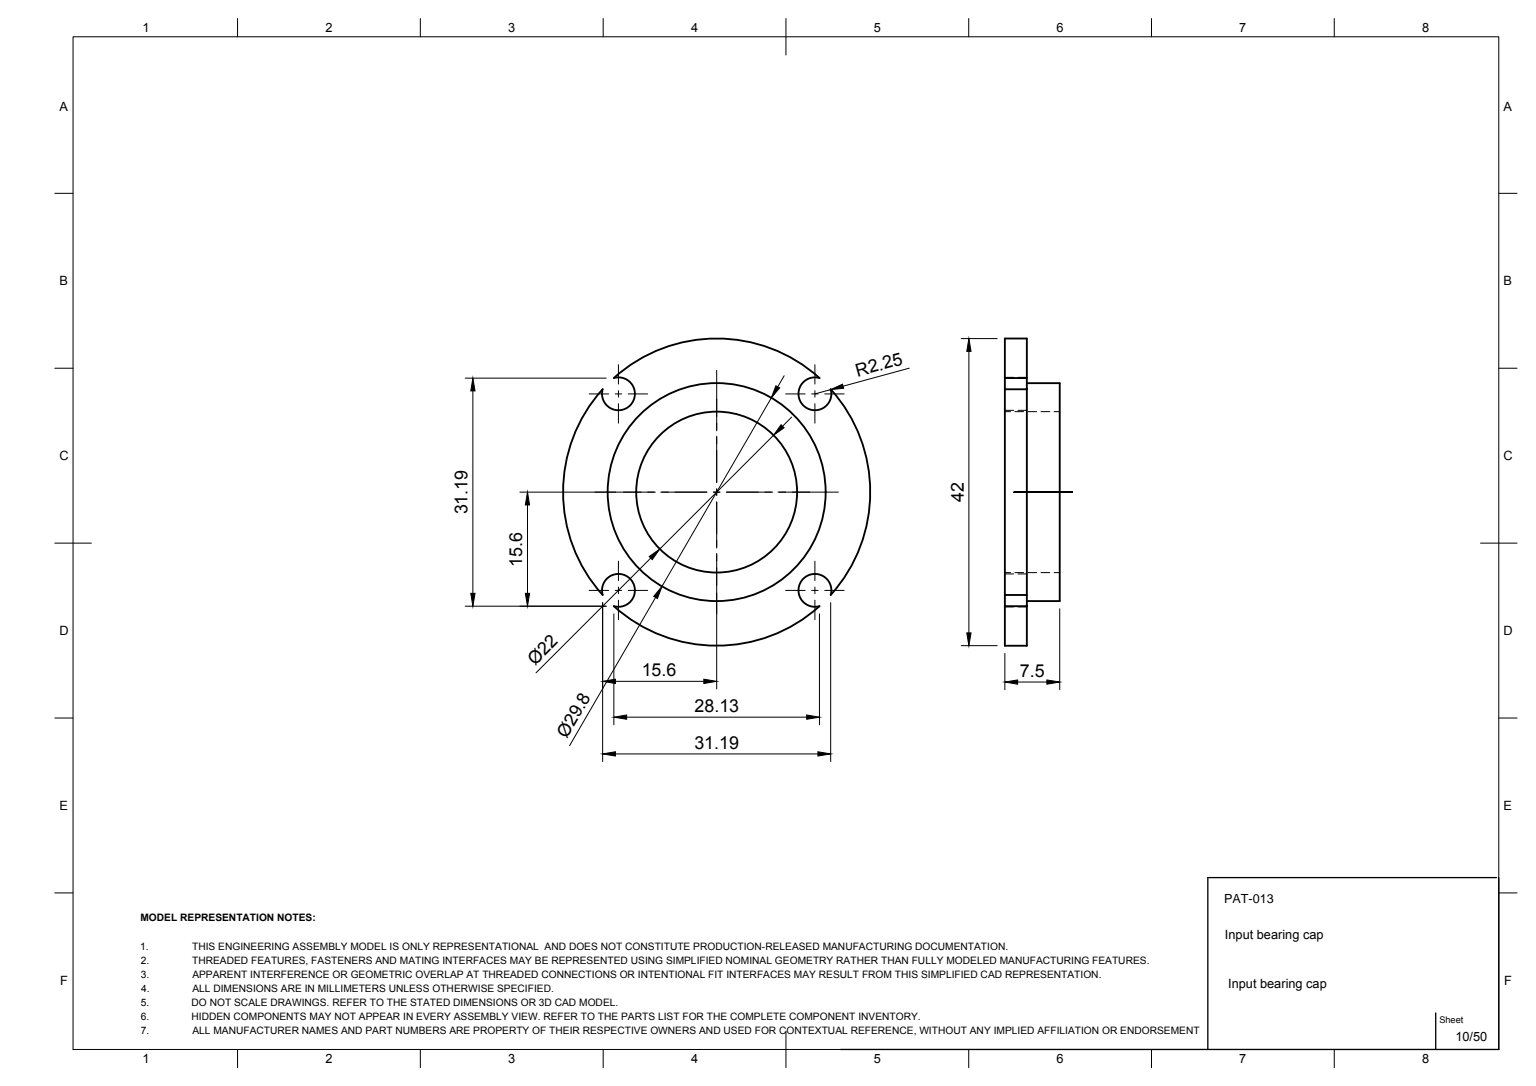
ISO-10303-21;
HEADER;
/* Generated by software containing ST-Developer
 * from STEP Tools, Inc. (www.steptools.com) 
 */

FILE_DESCRIPTION(
/* description */ ('Belt-driven linear axis on 2020 extrusion'),
/* implementation_level */ '2;1');

FILE_NAME(
/* name */ 'Input bearing cap.step',
/* time_stamp */ '2026-10-28T03:26:09-07:00',
/* author */ (''),
/* organization */ (''),
/* preprocessor_version */ 'ST-DEVELOPER v20.2',
/* originating_system */ 'Autodesk Translation Framework v15.17.0.0',
/* authorisation */ '');

FILE_SCHEMA (('AUTOMOTIVE_DESIGN { 1 0 10303 214 3 1 1 }'));
ENDSEC;

DATA;
#10=MECHANICAL_DESIGN_GEOMETRIC_PRESENTATION_REPRESENTATION('',(#617),#20096);
#523=SHAPE_REPRESENTATION_RELATIONSHIP('SRR','None',#20319,#569);
#569=ADVANCED_BREP_SHAPE_REPRESENTATION('',(#673),#20050);
#617=STYLED_ITEM('',(#20650),#673);
#673=MANIFOLD_SOLID_BREP('Body1',#10930);
#762=FACE_BOUND('',#2010,.T.);
#763=FACE_BOUND('',#2017,.T.);
#764=FACE_BOUND('',#2020,.T.);
#947=PLANE('',#11661);
#948=PLANE('',#11678);
#949=PLANE('',#11681);
#1339=FACE_OUTER_BOUND('',#2005,.T.);
#1340=FACE_OUTER_BOUND('',#2006,.T.);
#1341=FACE_OUTER_BOUND('',#2007,.T.);
#1342=FACE_OUTER_BOUND('',#2008,.T.);
#1343=FACE_OUTER_BOUND('',#2009,.T.);
#1344=FACE_OUTER_BOUND('',#2011,.T.);
#1345=FACE_OUTER_BOUND('',#2012,.T.);
#1346=FACE_OUTER_BOUND('',#2013,.T.);
#1347=FACE_OUTER_BOUND('',#2014,.T.);
#1348=FACE_OUTER_BOUND('',#2015,.T.);
#1349=FACE_OUTER_BOUND('',#2016,.T.);
#1350=FACE_OUTER_BOUND('',#2018,.T.);
#1351=FACE_OUTER_BOUND('',#2019,.T.);
#2005=EDGE_LOOP('',(#7607,#7608,#7609,#7610));
#2006=EDGE_LOOP('',(#7611,#7612,#7613,#7614));
#2007=EDGE_LOOP('',(#7615,#7616,#7617,#7618));
#2008=EDGE_LOOP('',(#7619,#7620,#7621,#7622));
#2009=EDGE_LOOP('',(#7623,#7624,#7625,#7626,#7627,#7628,#7629,#7630));
#2010=EDGE_LOOP('',(#7631));
#2011=EDGE_LOOP('',(#7632,#7633,#7634,#7635));
#2012=EDGE_LOOP('',(#7636,#7637,#7638,#7639));
#2013=EDGE_LOOP('',(#7640,#7641,#7642,#7643));
#2014=EDGE_LOOP('',(#7644,#7645,#7646,#7647));
#2015=EDGE_LOOP('',(#7648,#7649,#7650,#7651));
#2016=EDGE_LOOP('',(#7652));
#2017=EDGE_LOOP('',(#7653));
#2018=EDGE_LOOP('',(#7654,#7655,#7656,#7657));
#2019=EDGE_LOOP('',(#7658,#7659,#7660,#7661,#7662,#7663,#7664,#7665));
#2020=EDGE_LOOP('',(#7666));
#2780=LINE('',#16627,#3637);
#2781=LINE('',#16631,#3638);
#2782=LINE('',#16636,#3639);
#2783=LINE('',#16640,#3640);
#2784=LINE('',#16645,#3641);
#2785=LINE('',#16649,#3642);
#2786=LINE('',#16654,#3643);
#2787=LINE('',#16658,#3644);
#2788=LINE('',#16679,#3645);
#2789=LINE('',#16685,#3646);
#3637=VECTOR('',#13220,1.);
#3638=VECTOR('',#13223,1.);
#3639=VECTOR('',#13228,1.);
#3640=VECTOR('',#13231,1.);
#3641=VECTOR('',#13236,1.);
#3642=VECTOR('',#13239,1.);
#3643=VECTOR('',#13244,1.);
#3644=VECTOR('',#13247,1.);
#3645=VECTOR('',#13282,1.49);
#3646=VECTOR('',#13291,1.1);
#4441=CIRCLE('',#11650,0.225);
#4442=CIRCLE('',#11651,0.225);
#4443=CIRCLE('',#11653,0.225);
#4444=CIRCLE('',#11654,0.225);
#4445=CIRCLE('',#11656,0.225);
#4446=CIRCLE('',#11657,0.225);
#4447=CIRCLE('',#11659,0.225);
#4448=CIRCLE('',#11660,0.225);
#4449=CIRCLE('',#11662,2.1);
#4450=CIRCLE('',#11663,2.1);
#4451=CIRCLE('',#11664,2.1);
#4452=CIRCLE('',#11665,2.1);
#4453=CIRCLE('',#11666,1.1);
#4454=CIRCLE('',#11668,2.1);
#4455=CIRCLE('',#11670,2.1);
#4456=CIRCLE('',#11672,2.1);
#4457=CIRCLE('',#11674,2.1);
#4458=CIRCLE('',#11676,1.49);
#4459=CIRCLE('',#11677,1.49);
#4460=CIRCLE('',#11679,1.1);
#5010=VERTEX_POINT('',#16625);
#5011=VERTEX_POINT('',#16626);
#5012=VERTEX_POINT('',#16628);
#5013=VERTEX_POINT('',#16630);
#5014=VERTEX_POINT('',#16634);
#5015=VERTEX_POINT('',#16635);
#5016=VERTEX_POINT('',#16637);
#5017=VERTEX_POINT('',#16639);
#5018=VERTEX_POINT('',#16643);
#5019=VERTEX_POINT('',#16644);
#5020=VERTEX_POINT('',#16646);
#5021=VERTEX_POINT('',#16648);
#5022=VERTEX_POINT('',#16652);
#5023=VERTEX_POINT('',#16653);
#5024=VERTEX_POINT('',#16655);
#5025=VERTEX_POINT('',#16657);
#5026=VERTEX_POINT('',#16665);
#5027=VERTEX_POINT('',#16676);
#5028=VERTEX_POINT('',#16678);
#5029=VERTEX_POINT('',#16682);
#6018=EDGE_CURVE('',#5010,#5011,#2780,.T.);
#6019=EDGE_CURVE('',#5012,#5010,#4441,.T.);
#6020=EDGE_CURVE('',#5013,#5012,#2781,.T.);
#6021=EDGE_CURVE('',#5011,#5013,#4442,.T.);
#6022=EDGE_CURVE('',#5014,#5015,#2782,.T.);
#6023=EDGE_CURVE('',#5016,#5014,#4443,.T.);
#6024=EDGE_CURVE('',#5017,#5016,#2783,.T.);
#6025=EDGE_CURVE('',#5015,#5017,#4444,.T.);
#6026=EDGE_CURVE('',#5018,#5019,#2784,.T.);
#6027=EDGE_CURVE('',#5020,#5018,#4445,.T.);
#6028=EDGE_CURVE('',#5021,#5020,#2785,.T.);
#6029=EDGE_CURVE('',#5019,#5021,#4446,.T.);
#6030=EDGE_CURVE('',#5022,#5023,#2786,.T.);
#6031=EDGE_CURVE('',#5024,#5022,#4447,.T.);
#6032=EDGE_CURVE('',#5025,#5024,#2787,.T.);
#6033=EDGE_CURVE('',#5023,#5025,#4448,.T.);
#6034=EDGE_CURVE('',#5024,#5010,#4449,.T.);
#6035=EDGE_CURVE('',#5020,#5022,#4450,.T.);
#6036=EDGE_CURVE('',#5016,#5018,#4451,.T.);
#6037=EDGE_CURVE('',#5012,#5014,#4452,.T.);
#6038=EDGE_CURVE('',#5026,#5026,#4453,.T.);
#6039=EDGE_CURVE('',#5021,#5023,#4454,.T.);
#6040=EDGE_CURVE('',#5017,#5019,#4455,.T.);
#6041=EDGE_CURVE('',#5025,#5011,#4456,.T.);
#6042=EDGE_CURVE('',#5013,#5015,#4457,.T.);
#6043=EDGE_CURVE('',#5027,#5027,#4458,.T.);
#6044=EDGE_CURVE('',#5027,#5028,#2788,.T.);
#6045=EDGE_CURVE('',#5028,#5028,#4459,.T.);
#6046=EDGE_CURVE('',#5029,#5029,#4460,.T.);
#6047=EDGE_CURVE('',#5029,#5026,#2789,.T.);
#7607=ORIENTED_EDGE('',*,*,#6018,.F.);
#7608=ORIENTED_EDGE('',*,*,#6019,.F.);
#7609=ORIENTED_EDGE('',*,*,#6020,.F.);
#7610=ORIENTED_EDGE('',*,*,#6021,.F.);
#7611=ORIENTED_EDGE('',*,*,#6022,.F.);
#7612=ORIENTED_EDGE('',*,*,#6023,.F.);
#7613=ORIENTED_EDGE('',*,*,#6024,.F.);
#7614=ORIENTED_EDGE('',*,*,#6025,.F.);
#7615=ORIENTED_EDGE('',*,*,#6026,.F.);
#7616=ORIENTED_EDGE('',*,*,#6027,.F.);
#7617=ORIENTED_EDGE('',*,*,#6028,.F.);
#7618=ORIENTED_EDGE('',*,*,#6029,.F.);
#7619=ORIENTED_EDGE('',*,*,#6030,.F.);
#7620=ORIENTED_EDGE('',*,*,#6031,.F.);
#7621=ORIENTED_EDGE('',*,*,#6032,.F.);
#7622=ORIENTED_EDGE('',*,*,#6033,.F.);
#7623=ORIENTED_EDGE('',*,*,#6019,.T.);
#7624=ORIENTED_EDGE('',*,*,#6034,.F.);
#7625=ORIENTED_EDGE('',*,*,#6031,.T.);
#7626=ORIENTED_EDGE('',*,*,#6035,.F.);
#7627=ORIENTED_EDGE('',*,*,#6027,.T.);
#7628=ORIENTED_EDGE('',*,*,#6036,.F.);
#7629=ORIENTED_EDGE('',*,*,#6023,.T.);
#7630=ORIENTED_EDGE('',*,*,#6037,.F.);
#7631=ORIENTED_EDGE('',*,*,#6038,.F.);
#7632=ORIENTED_EDGE('',*,*,#6028,.T.);
#7633=ORIENTED_EDGE('',*,*,#6035,.T.);
#7634=ORIENTED_EDGE('',*,*,#6030,.T.);
#7635=ORIENTED_EDGE('',*,*,#6039,.F.);
#7636=ORIENTED_EDGE('',*,*,#6024,.T.);
#7637=ORIENTED_EDGE('',*,*,#6036,.T.);
#7638=ORIENTED_EDGE('',*,*,#6026,.T.);
#7639=ORIENTED_EDGE('',*,*,#6040,.F.);
#7640=ORIENTED_EDGE('',*,*,#6018,.T.);
#7641=ORIENTED_EDGE('',*,*,#6041,.F.);
#7642=ORIENTED_EDGE('',*,*,#6032,.T.);
#7643=ORIENTED_EDGE('',*,*,#6034,.T.);
#7644=ORIENTED_EDGE('',*,*,#6020,.T.);
#7645=ORIENTED_EDGE('',*,*,#6037,.T.);
#7646=ORIENTED_EDGE('',*,*,#6022,.T.);
#7647=ORIENTED_EDGE('',*,*,#6042,.F.);
#7648=ORIENTED_EDGE('',*,*,#6043,.F.);
#7649=ORIENTED_EDGE('',*,*,#6044,.T.);
#7650=ORIENTED_EDGE('',*,*,#6045,.F.);
#7651=ORIENTED_EDGE('',*,*,#6044,.F.);
#7652=ORIENTED_EDGE('',*,*,#6043,.T.);
#7653=ORIENTED_EDGE('',*,*,#6046,.T.);
#7654=ORIENTED_EDGE('',*,*,#6046,.F.);
#7655=ORIENTED_EDGE('',*,*,#6047,.T.);
#7656=ORIENTED_EDGE('',*,*,#6038,.T.);
#7657=ORIENTED_EDGE('',*,*,#6047,.F.);
#7658=ORIENTED_EDGE('',*,*,#6021,.T.);
#7659=ORIENTED_EDGE('',*,*,#6042,.T.);
#7660=ORIENTED_EDGE('',*,*,#6025,.T.);
#7661=ORIENTED_EDGE('',*,*,#6040,.T.);
#7662=ORIENTED_EDGE('',*,*,#6029,.T.);
#7663=ORIENTED_EDGE('',*,*,#6039,.T.);
#7664=ORIENTED_EDGE('',*,*,#6033,.T.);
#7665=ORIENTED_EDGE('',*,*,#6041,.T.);
#7666=ORIENTED_EDGE('',*,*,#6045,.T.);
#10108=CYLINDRICAL_SURFACE('',#11649,0.225);
#10109=CYLINDRICAL_SURFACE('',#11652,0.225);
#10110=CYLINDRICAL_SURFACE('',#11655,0.225);
#10111=CYLINDRICAL_SURFACE('',#11658,0.225);
#10112=CYLINDRICAL_SURFACE('',#11667,2.1);
#10113=CYLINDRICAL_SURFACE('',#11669,2.1);
#10114=CYLINDRICAL_SURFACE('',#11671,2.1);
#10115=CYLINDRICAL_SURFACE('',#11673,2.1);
#10116=CYLINDRICAL_SURFACE('',#11675,1.49);
#10117=CYLINDRICAL_SURFACE('',#11680,1.1);
#10390=ADVANCED_FACE('',(#1339),#10108,.F.);
#10391=ADVANCED_FACE('',(#1340),#10109,.F.);
#10392=ADVANCED_FACE('',(#1341),#10110,.F.);
#10393=ADVANCED_FACE('',(#1342),#10111,.F.);
#10394=ADVANCED_FACE('',(#1343,#762),#947,.F.);
#10395=ADVANCED_FACE('',(#1344),#10112,.T.);
#10396=ADVANCED_FACE('',(#1345),#10113,.T.);
#10397=ADVANCED_FACE('',(#1346),#10114,.T.);
#10398=ADVANCED_FACE('',(#1347),#10115,.T.);
#10399=ADVANCED_FACE('',(#1348),#10116,.T.);
#10400=ADVANCED_FACE('',(#1349,#763),#948,.T.);
#10401=ADVANCED_FACE('',(#1350),#10117,.F.);
#10402=ADVANCED_FACE('',(#1351,#764),#949,.T.);
#10930=CLOSED_SHELL('',(#10390,#10391,#10392,#10393,#10394,#10395,#10396,
#10397,#10398,#10399,#10400,#10401,#10402));
#11648=AXIS2_PLACEMENT_3D('',#16623,#13216,#13217);
#11649=AXIS2_PLACEMENT_3D('',#16624,#13218,#13219);
#11650=AXIS2_PLACEMENT_3D('',#16629,#13221,#13222);
#11651=AXIS2_PLACEMENT_3D('',#16632,#13224,#13225);
#11652=AXIS2_PLACEMENT_3D('',#16633,#13226,#13227);
#11653=AXIS2_PLACEMENT_3D('',#16638,#13229,#13230);
#11654=AXIS2_PLACEMENT_3D('',#16641,#13232,#13233);
#11655=AXIS2_PLACEMENT_3D('',#16642,#13234,#13235);
#11656=AXIS2_PLACEMENT_3D('',#16647,#13237,#13238);
#11657=AXIS2_PLACEMENT_3D('',#16650,#13240,#13241);
#11658=AXIS2_PLACEMENT_3D('',#16651,#13242,#13243);
#11659=AXIS2_PLACEMENT_3D('',#16656,#13245,#13246);
#11660=AXIS2_PLACEMENT_3D('',#16659,#13248,#13249);
#11661=AXIS2_PLACEMENT_3D('',#16660,#13250,#13251);
#11662=AXIS2_PLACEMENT_3D('',#16661,#13252,#13253);
#11663=AXIS2_PLACEMENT_3D('',#16662,#13254,#13255);
#11664=AXIS2_PLACEMENT_3D('',#16663,#13256,#13257);
#11665=AXIS2_PLACEMENT_3D('',#16664,#13258,#13259);
#11666=AXIS2_PLACEMENT_3D('',#16666,#13260,#13261);
#11667=AXIS2_PLACEMENT_3D('',#16667,#13262,#13263);
#11668=AXIS2_PLACEMENT_3D('',#16668,#13264,#13265);
#11669=AXIS2_PLACEMENT_3D('',#16669,#13266,#13267);
#11670=AXIS2_PLACEMENT_3D('',#16670,#13268,#13269);
#11671=AXIS2_PLACEMENT_3D('',#16671,#13270,#13271);
#11672=AXIS2_PLACEMENT_3D('',#16672,#13272,#13273);
#11673=AXIS2_PLACEMENT_3D('',#16673,#13274,#13275);
#11674=AXIS2_PLACEMENT_3D('',#16674,#13276,#13277);
#11675=AXIS2_PLACEMENT_3D('',#16675,#13278,#13279);
#11676=AXIS2_PLACEMENT_3D('',#16677,#13280,#13281);
#11677=AXIS2_PLACEMENT_3D('',#16680,#13283,#13284);
#11678=AXIS2_PLACEMENT_3D('',#16681,#13285,#13286);
#11679=AXIS2_PLACEMENT_3D('',#16683,#13287,#13288);
#11680=AXIS2_PLACEMENT_3D('',#16684,#13289,#13290);
#11681=AXIS2_PLACEMENT_3D('',#16686,#13292,#13293);
#13216=DIRECTION('axis',(0.,0.,1.));
#13217=DIRECTION('refdir',(1.,0.,0.));
#13218=DIRECTION('center_axis',(0.,1.,0.));
#13219=DIRECTION('ref_axis',(0.707106781186546,0.,0.707106781186549));
#13220=DIRECTION('',(0.,1.,0.));
#13221=DIRECTION('center_axis',(0.,1.,0.));
#13222=DIRECTION('ref_axis',(1.,0.,0.));
#13223=DIRECTION('',(0.,-1.,0.));
#13224=DIRECTION('center_axis',(0.,-1.,0.));
#13225=DIRECTION('ref_axis',(1.,0.,0.));
#13226=DIRECTION('center_axis',(0.,1.,0.));
#13227=DIRECTION('ref_axis',(0.707106781186547,0.,-0.707106781186548));
#13228=DIRECTION('',(0.,1.,0.));
#13229=DIRECTION('center_axis',(0.,1.,0.));
#13230=DIRECTION('ref_axis',(1.,0.,0.));
#13231=DIRECTION('',(0.,-1.,0.));
#13232=DIRECTION('center_axis',(0.,-1.,0.));
#13233=DIRECTION('ref_axis',(1.,0.,0.));
#13234=DIRECTION('center_axis',(0.,1.,0.));
#13235=DIRECTION('ref_axis',(-0.707106781186552,0.,-0.707106781186543));
#13236=DIRECTION('',(0.,1.,0.));
#13237=DIRECTION('center_axis',(0.,1.,0.));
#13238=DIRECTION('ref_axis',(1.,0.,0.));
#13239=DIRECTION('',(0.,-1.,0.));
#13240=DIRECTION('center_axis',(0.,-1.,0.));
#13241=DIRECTION('ref_axis',(1.,0.,0.));
#13242=DIRECTION('center_axis',(0.,1.,0.));
#13243=DIRECTION('ref_axis',(-0.707106781186546,0.,0.707106781186549));
#13244=DIRECTION('',(0.,1.,0.));
#13245=DIRECTION('center_axis',(0.,1.,0.));
#13246=DIRECTION('ref_axis',(1.,0.,0.));
#13247=DIRECTION('',(0.,-1.,0.));
#13248=DIRECTION('center_axis',(0.,-1.,0.));
#13249=DIRECTION('ref_axis',(1.,0.,0.));
#13250=DIRECTION('center_axis',(0.,1.,0.));
#13251=DIRECTION('ref_axis',(1.,0.,0.));
#13252=DIRECTION('center_axis',(0.,1.,0.));
#13253=DIRECTION('ref_axis',(1.,0.,0.));
#13254=DIRECTION('center_axis',(0.,1.,0.));
#13255=DIRECTION('ref_axis',(1.,0.,0.));
#13256=DIRECTION('center_axis',(0.,1.,0.));
#13257=DIRECTION('ref_axis',(1.,0.,0.));
#13258=DIRECTION('center_axis',(0.,1.,0.));
#13259=DIRECTION('ref_axis',(1.,0.,0.));
#13260=DIRECTION('center_axis',(0.,-1.,0.));
#13261=DIRECTION('ref_axis',(1.,0.,0.));
#13262=DIRECTION('center_axis',(0.,1.,0.));
#13263=DIRECTION('ref_axis',(1.,0.,0.));
#13264=DIRECTION('center_axis',(0.,1.,0.));
#13265=DIRECTION('ref_axis',(1.,0.,0.));
#13266=DIRECTION('center_axis',(0.,1.,0.));
#13267=DIRECTION('ref_axis',(1.,0.,0.));
#13268=DIRECTION('center_axis',(0.,1.,0.));
#13269=DIRECTION('ref_axis',(1.,0.,0.));
#13270=DIRECTION('center_axis',(0.,1.,0.));
#13271=DIRECTION('ref_axis',(1.,0.,0.));
#13272=DIRECTION('center_axis',(0.,1.,0.));
#13273=DIRECTION('ref_axis',(1.,0.,0.));
#13274=DIRECTION('center_axis',(0.,1.,0.));
#13275=DIRECTION('ref_axis',(-1.,0.,-1.22464679914735E-16));
#13276=DIRECTION('center_axis',(0.,1.,0.));
#13277=DIRECTION('ref_axis',(1.,0.,0.));
#13278=DIRECTION('center_axis',(0.,1.,0.));
#13279=DIRECTION('ref_axis',(1.,0.,0.));
#13280=DIRECTION('center_axis',(0.,1.,0.));
#13281=DIRECTION('ref_axis',(1.,0.,0.));
#13282=DIRECTION('',(0.,-1.,0.));
#13283=DIRECTION('center_axis',(0.,-1.,0.));
#13284=DIRECTION('ref_axis',(1.,0.,0.));
#13285=DIRECTION('center_axis',(0.,1.,0.));
#13286=DIRECTION('ref_axis',(1.,0.,0.));
#13287=DIRECTION('center_axis',(0.,-1.,0.));
#13288=DIRECTION('ref_axis',(1.,0.,0.));
#13289=DIRECTION('center_axis',(0.,1.,0.));
#13290=DIRECTION('ref_axis',(1.,0.,0.));
#13291=DIRECTION('',(0.,-1.,0.));
#13292=DIRECTION('center_axis',(0.,1.,0.));
#13293=DIRECTION('ref_axis',(1.,0.,0.));
#16623=CARTESIAN_POINT('',(0.,0.,0.));
#16624=CARTESIAN_POINT('Origin',(-1.34350288425444,-2.2,5.65649711574556));
#16625=CARTESIAN_POINT('',(-1.40634555589641,-2.1,5.4404512904656));
#16626=CARTESIAN_POINT('',(-1.40634555589641,-1.8,5.4404512904656));
#16627=CARTESIAN_POINT('',(-1.40634555589641,-2.2,5.4404512904656));
#16628=CARTESIAN_POINT('',(-1.5595487095344,-2.1,5.59365444410359));
#16629=CARTESIAN_POINT('Origin',(-1.34350288425444,-2.1,5.65649711574556));
#16630=CARTESIAN_POINT('',(-1.5595487095344,-1.8,5.59365444410359));
#16631=CARTESIAN_POINT('',(-1.5595487095344,-2.2,5.59365444410359));
#16632=CARTESIAN_POINT('Origin',(-1.34350288425444,-1.8,5.65649711574556));
#16633=CARTESIAN_POINT('Origin',(-1.34350288425444,-2.2,8.34350288425444));
#16634=CARTESIAN_POINT('',(-1.5595487095344,-2.1,8.40634555589641));
#16635=CARTESIAN_POINT('',(-1.5595487095344,-1.8,8.40634555589641));
#16636=CARTESIAN_POINT('',(-1.5595487095344,-2.2,8.40634555589641));
#16637=CARTESIAN_POINT('',(-1.40634555589641,-2.1,8.5595487095344));
#16638=CARTESIAN_POINT('Origin',(-1.34350288425444,-2.1,8.34350288425444));
#16639=CARTESIAN_POINT('',(-1.40634555589641,-1.8,8.5595487095344));
#16640=CARTESIAN_POINT('',(-1.40634555589641,-2.2,8.5595487095344));
#16641=CARTESIAN_POINT('Origin',(-1.34350288425444,-1.8,8.34350288425444));
#16642=CARTESIAN_POINT('Origin',(1.34350288425444,-2.2,8.34350288425444));
#16643=CARTESIAN_POINT('',(1.40634555589641,-2.1,8.5595487095344));
#16644=CARTESIAN_POINT('',(1.40634555589641,-1.8,8.5595487095344));
#16645=CARTESIAN_POINT('',(1.40634555589641,-2.2,8.5595487095344));
#16646=CARTESIAN_POINT('',(1.5595487095344,-2.1,8.40634555589641));
#16647=CARTESIAN_POINT('Origin',(1.34350288425444,-2.1,8.34350288425444));
#16648=CARTESIAN_POINT('',(1.5595487095344,-1.8,8.40634555589641));
#16649=CARTESIAN_POINT('',(1.5595487095344,-2.2,8.40634555589641));
#16650=CARTESIAN_POINT('Origin',(1.34350288425444,-1.8,8.34350288425444));
#16651=CARTESIAN_POINT('Origin',(1.34350288425444,-2.2,5.65649711574556));
#16652=CARTESIAN_POINT('',(1.5595487095344,-2.1,5.59365444410359));
#16653=CARTESIAN_POINT('',(1.5595487095344,-1.8,5.59365444410359));
#16654=CARTESIAN_POINT('',(1.5595487095344,-2.2,5.59365444410359));
#16655=CARTESIAN_POINT('',(1.40634555589641,-2.1,5.4404512904656));
#16656=CARTESIAN_POINT('Origin',(1.34350288425444,-2.1,5.65649711574556));
#16657=CARTESIAN_POINT('',(1.40634555589641,-1.8,5.4404512904656));
#16658=CARTESIAN_POINT('',(1.40634555589641,-2.2,5.4404512904656));
#16659=CARTESIAN_POINT('Origin',(1.34350288425444,-1.8,5.65649711574556));
#16660=CARTESIAN_POINT('Origin',(0.,-2.1,7.));
#16661=CARTESIAN_POINT('Origin',(0.,-2.1,7.));
#16662=CARTESIAN_POINT('Origin',(0.,-2.1,7.));
#16663=CARTESIAN_POINT('Origin',(0.,-2.1,7.));
#16664=CARTESIAN_POINT('Origin',(0.,-2.1,7.));
#16665=CARTESIAN_POINT('',(-1.1,-2.1,7.));
#16666=CARTESIAN_POINT('Origin',(0.,-2.1,7.));
#16667=CARTESIAN_POINT('Origin',(0.,-2.1,7.));
#16668=CARTESIAN_POINT('Origin',(0.,-1.8,7.));
#16669=CARTESIAN_POINT('Origin',(0.,-2.1,7.));
#16670=CARTESIAN_POINT('Origin',(0.,-1.8,7.));
#16671=CARTESIAN_POINT('Origin',(0.,-2.1,7.));
#16672=CARTESIAN_POINT('Origin',(0.,-1.8,7.));
#16673=CARTESIAN_POINT('Origin',(0.,-2.1,7.));
#16674=CARTESIAN_POINT('Origin',(0.,-1.8,7.));
#16675=CARTESIAN_POINT('Origin',(0.,-1.8,7.));
#16676=CARTESIAN_POINT('',(-1.49,-1.35,7.));
#16677=CARTESIAN_POINT('Origin',(0.,-1.35,7.));
#16678=CARTESIAN_POINT('',(-1.49,-1.8,7.));
#16679=CARTESIAN_POINT('',(-1.49,-1.8,7.));
#16680=CARTESIAN_POINT('Origin',(0.,-1.8,7.));
#16681=CARTESIAN_POINT('Origin',(0.,-1.35,7.));
#16682=CARTESIAN_POINT('',(-1.1,-1.35,7.));
#16683=CARTESIAN_POINT('Origin',(0.,-1.35,7.));
#16684=CARTESIAN_POINT('Origin',(0.,-2.1,7.));
#16685=CARTESIAN_POINT('',(-1.1,-2.1,7.));
#16686=CARTESIAN_POINT('Origin',(0.,-1.8,7.));
#19996=UNCERTAINTY_MEASURE_WITH_UNIT(LENGTH_MEASURE(0.001),#20097,
'DISTANCE_ACCURACY_VALUE',
'Maximum model space distance between geometric entities at asserted c
onnectivities');
#20042=UNCERTAINTY_MEASURE_WITH_UNIT(LENGTH_MEASURE(0.001),#20097,
'DISTANCE_ACCURACY_VALUE',
'Maximum model space distance between geometric entities at asserted c
onnectivities');
#20050=(
GEOMETRIC_REPRESENTATION_CONTEXT(3)
GLOBAL_UNCERTAINTY_ASSIGNED_CONTEXT((#19996))
GLOBAL_UNIT_ASSIGNED_CONTEXT((#20097,#20099,#20100))
REPRESENTATION_CONTEXT('','3D')
);
#20096=(
GEOMETRIC_REPRESENTATION_CONTEXT(3)
GLOBAL_UNCERTAINTY_ASSIGNED_CONTEXT((#20042))
GLOBAL_UNIT_ASSIGNED_CONTEXT((#20097,#20099,#20100))
REPRESENTATION_CONTEXT('','3D')
);
#20097=(
LENGTH_UNIT()
NAMED_UNIT(*)
SI_UNIT(.CENTI.,.METRE.)
);
#20099=(
NAMED_UNIT(*)
PLANE_ANGLE_UNIT()
SI_UNIT($,.RADIAN.)
);
#20100=(
NAMED_UNIT(*)
SI_UNIT($,.STERADIAN.)
SOLID_ANGLE_UNIT()
);
#20108=SHAPE_DEFINITION_REPRESENTATION(#20161,#20319);
#20161=PRODUCT_DEFINITION_SHAPE('',$,#20373);
#20319=SHAPE_REPRESENTATION('',(#11648),#20050);
#20365=PRODUCT_DEFINITION_CONTEXT('part definition',#20526,'design');
#20373=PRODUCT_DEFINITION('Input bearing cap','Input bearing cap',#20426,
#20365);
#20426=PRODUCT_DEFINITION_FORMATION('',$,#20535);
#20526=APPLICATION_CONTEXT(
'Core Data for Automotive Mechanical Design Process');
#20527=PRODUCT_CONTEXT('part definition',#20526,'mechanical');
#20535=PRODUCT('Input bearing cap','Input bearing cap',
'Input bearing cap',(#20527));
#20644=COLOUR_RGB('Grey',0.48,0.52,0.57);
#20645=FILL_AREA_STYLE_COLOUR('',#20644);
#20646=FILL_AREA_STYLE('',(#20645));
#20647=SURFACE_STYLE_FILL_AREA(#20646);
#20648=SURFACE_SIDE_STYLE('',(#20647));
#20649=SURFACE_STYLE_USAGE(.BOTH.,#20648);
#20650=PRESENTATION_STYLE_ASSIGNMENT((#20649));
ENDSEC;
END-ISO-10303-21;
